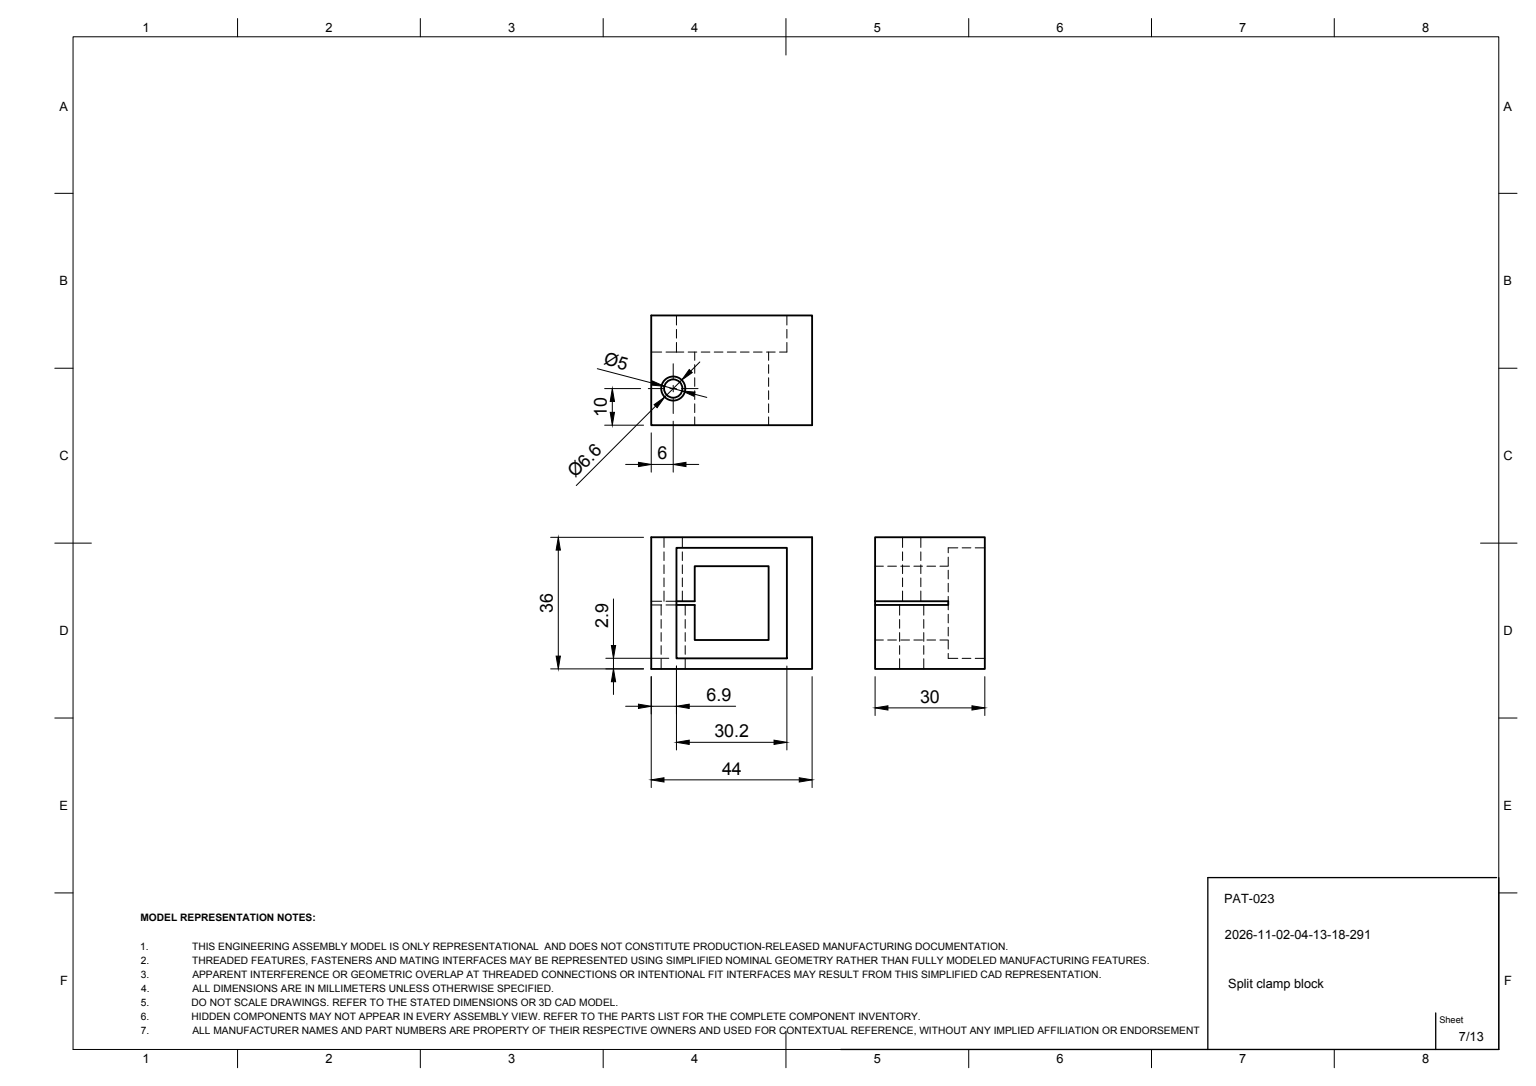
ISO-10303-21;
HEADER;
/* Generated by software containing ST-Developer
 * from STEP Tools, Inc. (www.steptools.com) 
 */

FILE_DESCRIPTION(
/* description */ ('PAT-023'),
/* implementation_level */ '2;1');

FILE_NAME(
/* name */ 'Split clamp block.step',
/* time_stamp */ '2026-10-29T15:47:46-07:00',
/* author */ (''),
/* organization */ (''),
/* preprocessor_version */ 'ST-DEVELOPER v20.2',
/* originating_system */ 'Autodesk Translation Framework v15.17.0.0',
/* authorisation */ '');

FILE_SCHEMA (('AUTOMOTIVE_DESIGN { 1 0 10303 214 3 1 1 }'));
ENDSEC;

DATA;
#10=MECHANICAL_DESIGN_GEOMETRIC_PRESENTATION_REPRESENTATION('',(#86),#3773);
#70=SHAPE_REPRESENTATION_RELATIONSHIP('SRR','None',#3817,#78);
#78=ADVANCED_BREP_SHAPE_REPRESENTATION('',(#94),#3765);
#86=STYLED_ITEM('',(#3925),#94);
#94=MANIFOLD_SOLID_BREP('Body1',#2239);
#104=FACE_BOUND('',#361,.T.);
#105=FACE_BOUND('',#363,.T.);
#106=FACE_BOUND('',#378,.T.);
#107=FACE_BOUND('',#380,.T.);
#108=FACE_BOUND('',#383,.T.);
#131=PLANE('',#2364);
#132=PLANE('',#2365);
#133=PLANE('',#2366);
#134=PLANE('',#2367);
#135=PLANE('',#2368);
#136=PLANE('',#2369);
#137=PLANE('',#2370);
#138=PLANE('',#2371);
#139=PLANE('',#2372);
#140=PLANE('',#2373);
#141=PLANE('',#2374);
#142=PLANE('',#2375);
#143=PLANE('',#2376);
#144=PLANE('',#2377);
#145=PLANE('',#2378);
#146=PLANE('',#2379);
#147=PLANE('',#2380);
#148=PLANE('',#2381);
#149=PLANE('',#2382);
#235=FACE_OUTER_BOUND('',#358,.T.);
#236=FACE_OUTER_BOUND('',#359,.T.);
#237=FACE_OUTER_BOUND('',#360,.T.);
#238=FACE_OUTER_BOUND('',#362,.T.);
#239=FACE_OUTER_BOUND('',#364,.T.);
#240=FACE_OUTER_BOUND('',#365,.T.);
#241=FACE_OUTER_BOUND('',#366,.T.);
#242=FACE_OUTER_BOUND('',#367,.T.);
#243=FACE_OUTER_BOUND('',#368,.T.);
#244=FACE_OUTER_BOUND('',#369,.T.);
#245=FACE_OUTER_BOUND('',#370,.T.);
#246=FACE_OUTER_BOUND('',#371,.T.);
#247=FACE_OUTER_BOUND('',#372,.T.);
#248=FACE_OUTER_BOUND('',#373,.T.);
#249=FACE_OUTER_BOUND('',#374,.T.);
#250=FACE_OUTER_BOUND('',#375,.T.);
#251=FACE_OUTER_BOUND('',#376,.T.);
#252=FACE_OUTER_BOUND('',#377,.T.);
#253=FACE_OUTER_BOUND('',#379,.T.);
#254=FACE_OUTER_BOUND('',#381,.T.);
#255=FACE_OUTER_BOUND('',#382,.T.);
#358=EDGE_LOOP('',(#1595,#1596,#1597,#1598));
#359=EDGE_LOOP('',(#1599,#1600,#1601,#1602));
#360=EDGE_LOOP('',(#1603,#1604,#1605,#1606,#1607));
#361=EDGE_LOOP('',(#1608));
#362=EDGE_LOOP('',(#1609,#1610,#1611,#1612,#1613));
#363=EDGE_LOOP('',(#1614));
#364=EDGE_LOOP('',(#1615,#1616,#1617,#1618));
#365=EDGE_LOOP('',(#1619,#1620,#1621,#1622,#1623,#1624,#1625,#1626,#1627,
#1628,#1629,#1630));
#366=EDGE_LOOP('',(#1631,#1632,#1633,#1634));
#367=EDGE_LOOP('',(#1635,#1636,#1637,#1638));
#368=EDGE_LOOP('',(#1639,#1640,#1641,#1642,#1643,#1644,#1645,#1646));
#369=EDGE_LOOP('',(#1647,#1648,#1649,#1650,#1651,#1652,#1653,#1654,#1655,
#1656,#1657,#1658));
#370=EDGE_LOOP('',(#1659,#1660,#1661,#1662));
#371=EDGE_LOOP('',(#1663,#1664,#1665,#1666));
#372=EDGE_LOOP('',(#1667,#1668,#1669,#1670));
#373=EDGE_LOOP('',(#1671,#1672,#1673,#1674));
#374=EDGE_LOOP('',(#1675,#1676,#1677,#1678,#1679,#1680));
#375=EDGE_LOOP('',(#1681,#1682,#1683,#1684));
#376=EDGE_LOOP('',(#1685,#1686,#1687,#1688));
#377=EDGE_LOOP('',(#1689,#1690,#1691,#1692));
#378=EDGE_LOOP('',(#1693));
#379=EDGE_LOOP('',(#1694,#1695,#1696,#1697));
#380=EDGE_LOOP('',(#1698));
#381=EDGE_LOOP('',(#1699,#1700,#1701,#1702));
#382=EDGE_LOOP('',(#1703,#1704,#1705,#1706));
#383=EDGE_LOOP('',(#1707,#1708,#1709,#1710));
#508=LINE('',#3193,#772);
#509=LINE('',#3199,#773);
#510=LINE('',#3204,#774);
#511=LINE('',#3206,#775);
#512=LINE('',#3208,#776);
#513=LINE('',#3210,#777);
#514=LINE('',#3211,#778);
#515=LINE('',#3215,#779);
#516=LINE('',#3217,#780);
#517=LINE('',#3219,#781);
#518=LINE('',#3221,#782);
#519=LINE('',#3222,#783);
#520=LINE('',#3224,#784);
#521=LINE('',#3225,#785);
#522=LINE('',#3228,#786);
#523=LINE('',#3230,#787);
#524=LINE('',#3232,#788);
#525=LINE('',#3234,#789);
#526=LINE('',#3235,#790);
#527=LINE('',#3237,#791);
#528=LINE('',#3239,#792);
#529=LINE('',#3241,#793);
#530=LINE('',#3243,#794);
#531=LINE('',#3244,#795);
#532=LINE('',#3247,#796);
#533=LINE('',#3248,#797);
#534=LINE('',#3251,#798);
#535=LINE('',#3252,#799);
#536=LINE('',#3255,#800);
#537=LINE('',#3257,#801);
#538=LINE('',#3259,#802);
#539=LINE('',#3261,#803);
#540=LINE('',#3262,#804);
#541=LINE('',#3265,#805);
#542=LINE('',#3267,#806);
#543=LINE('',#3268,#807);
#544=LINE('',#3270,#808);
#545=LINE('',#3272,#809);
#546=LINE('',#3273,#810);
#547=LINE('',#3275,#811);
#548=LINE('',#3277,#812);
#549=LINE('',#3282,#813);
#550=LINE('',#3283,#814);
#551=LINE('',#3284,#815);
#552=LINE('',#3287,#816);
#553=LINE('',#3288,#817);
#554=LINE('',#3291,#818);
#555=LINE('',#3292,#819);
#556=LINE('',#3294,#820);
#557=LINE('',#3297,#821);
#558=LINE('',#3298,#822);
#559=LINE('',#3301,#823);
#560=LINE('',#3302,#824);
#561=LINE('',#3304,#825);
#772=VECTOR('',#2591,0.25);
#773=VECTOR('',#2598,0.33);
#774=VECTOR('',#2603,1.);
#775=VECTOR('',#2604,1.);
#776=VECTOR('',#2605,1.);
#777=VECTOR('',#2606,1.);
#778=VECTOR('',#2607,1.);
#779=VECTOR('',#2610,1.);
#780=VECTOR('',#2611,1.);
#781=VECTOR('',#2612,1.);
#782=VECTOR('',#2613,1.);
#783=VECTOR('',#2614,1.);
#784=VECTOR('',#2617,1.);
#785=VECTOR('',#2618,1.);
#786=VECTOR('',#2621,1.);
#787=VECTOR('',#2622,1.);
#788=VECTOR('',#2623,1.);
#789=VECTOR('',#2624,1.);
#790=VECTOR('',#2625,1.);
#791=VECTOR('',#2626,1.);
#792=VECTOR('',#2627,1.);
#793=VECTOR('',#2628,1.);
#794=VECTOR('',#2629,1.);
#795=VECTOR('',#2630,1.);
#796=VECTOR('',#2633,1.);
#797=VECTOR('',#2634,1.);
#798=VECTOR('',#2637,1.);
#799=VECTOR('',#2638,1.);
#800=VECTOR('',#2641,1.);
#801=VECTOR('',#2642,1.);
#802=VECTOR('',#2643,1.);
#803=VECTOR('',#2644,1.);
#804=VECTOR('',#2645,1.);
#805=VECTOR('',#2648,1.);
#806=VECTOR('',#2649,1.);
#807=VECTOR('',#2650,1.);
#808=VECTOR('',#2651,1.);
#809=VECTOR('',#2652,1.);
#810=VECTOR('',#2653,1.);
#811=VECTOR('',#2656,1.);
#812=VECTOR('',#2659,1.);
#813=VECTOR('',#2664,1.);
#814=VECTOR('',#2665,1.);
#815=VECTOR('',#2666,1.);
#816=VECTOR('',#2669,1.);
#817=VECTOR('',#2670,1.);
#818=VECTOR('',#2673,1.);
#819=VECTOR('',#2674,1.);
#820=VECTOR('',#2677,1.);
#821=VECTOR('',#2680,1.);
#822=VECTOR('',#2681,1.);
#823=VECTOR('',#2684,1.);
#824=VECTOR('',#2685,1.);
#825=VECTOR('',#2688,1.);
#1001=CIRCLE('',#2359,0.25);
#1002=CIRCLE('',#2360,0.25);
#1003=CIRCLE('',#2362,0.33);
#1004=CIRCLE('',#2363,0.33);
#1051=VERTEX_POINT('',#3190);
#1052=VERTEX_POINT('',#3192);
#1053=VERTEX_POINT('',#3196);
#1054=VERTEX_POINT('',#3198);
#1055=VERTEX_POINT('',#3202);
#1056=VERTEX_POINT('',#3203);
#1057=VERTEX_POINT('',#3205);
#1058=VERTEX_POINT('',#3207);
#1059=VERTEX_POINT('',#3209);
#1060=VERTEX_POINT('',#3213);
#1061=VERTEX_POINT('',#3214);
#1062=VERTEX_POINT('',#3216);
#1063=VERTEX_POINT('',#3218);
#1064=VERTEX_POINT('',#3220);
#1065=VERTEX_POINT('',#3227);
#1066=VERTEX_POINT('',#3229);
#1067=VERTEX_POINT('',#3231);
#1068=VERTEX_POINT('',#3233);
#1069=VERTEX_POINT('',#3236);
#1070=VERTEX_POINT('',#3238);
#1071=VERTEX_POINT('',#3240);
#1072=VERTEX_POINT('',#3242);
#1073=VERTEX_POINT('',#3246);
#1074=VERTEX_POINT('',#3250);
#1075=VERTEX_POINT('',#3254);
#1076=VERTEX_POINT('',#3256);
#1077=VERTEX_POINT('',#3258);
#1078=VERTEX_POINT('',#3260);
#1079=VERTEX_POINT('',#3264);
#1080=VERTEX_POINT('',#3266);
#1081=VERTEX_POINT('',#3269);
#1082=VERTEX_POINT('',#3271);
#1083=VERTEX_POINT('',#3280);
#1084=VERTEX_POINT('',#3281);
#1085=VERTEX_POINT('',#3286);
#1086=VERTEX_POINT('',#3290);
#1087=VERTEX_POINT('',#3296);
#1088=VERTEX_POINT('',#3300);
#1260=EDGE_CURVE('',#1051,#1051,#1001,.T.);
#1261=EDGE_CURVE('',#1051,#1052,#508,.T.);
#1262=EDGE_CURVE('',#1052,#1052,#1002,.T.);
#1263=EDGE_CURVE('',#1053,#1053,#1003,.T.);
#1264=EDGE_CURVE('',#1053,#1054,#509,.T.);
#1265=EDGE_CURVE('',#1054,#1054,#1004,.T.);
#1266=EDGE_CURVE('',#1055,#1056,#510,.T.);
#1267=EDGE_CURVE('',#1057,#1055,#511,.T.);
#1268=EDGE_CURVE('',#1058,#1057,#512,.T.);
#1269=EDGE_CURVE('',#1059,#1058,#513,.T.);
#1270=EDGE_CURVE('',#1056,#1059,#514,.T.);
#1271=EDGE_CURVE('',#1060,#1061,#515,.T.);
#1272=EDGE_CURVE('',#1062,#1060,#516,.T.);
#1273=EDGE_CURVE('',#1063,#1062,#517,.T.);
#1274=EDGE_CURVE('',#1064,#1063,#518,.T.);
#1275=EDGE_CURVE('',#1061,#1064,#519,.T.);
#1276=EDGE_CURVE('',#1064,#1057,#520,.T.);
#1277=EDGE_CURVE('',#1058,#1063,#521,.T.);
#1278=EDGE_CURVE('',#1055,#1065,#522,.T.);
#1279=EDGE_CURVE('',#1065,#1066,#523,.T.);
#1280=EDGE_CURVE('',#1066,#1067,#524,.T.);
#1281=EDGE_CURVE('',#1067,#1068,#525,.T.);
#1282=EDGE_CURVE('',#1068,#1061,#526,.T.);
#1283=EDGE_CURVE('',#1069,#1064,#527,.T.);
#1284=EDGE_CURVE('',#1070,#1069,#528,.T.);
#1285=EDGE_CURVE('',#1071,#1070,#529,.T.);
#1286=EDGE_CURVE('',#1072,#1071,#530,.T.);
#1287=EDGE_CURVE('',#1057,#1072,#531,.T.);
#1288=EDGE_CURVE('',#1068,#1073,#532,.T.);
#1289=EDGE_CURVE('',#1060,#1073,#533,.T.);
#1290=EDGE_CURVE('',#1074,#1056,#534,.T.);
#1291=EDGE_CURVE('',#1065,#1074,#535,.T.);
#1292=EDGE_CURVE('',#1075,#1062,#536,.T.);
#1293=EDGE_CURVE('',#1076,#1075,#537,.T.);
#1294=EDGE_CURVE('',#1076,#1077,#538,.T.);
#1295=EDGE_CURVE('',#1077,#1078,#539,.T.);
#1296=EDGE_CURVE('',#1059,#1078,#540,.T.);
#1297=EDGE_CURVE('',#1078,#1079,#541,.T.);
#1298=EDGE_CURVE('',#1079,#1080,#542,.T.);
#1299=EDGE_CURVE('',#1080,#1075,#543,.T.);
#1300=EDGE_CURVE('',#1073,#1081,#544,.T.);
#1301=EDGE_CURVE('',#1081,#1082,#545,.T.);
#1302=EDGE_CURVE('',#1082,#1074,#546,.T.);
#1303=EDGE_CURVE('',#1067,#1081,#547,.T.);
#1304=EDGE_CURVE('',#1066,#1082,#548,.T.);
#1305=EDGE_CURVE('',#1083,#1084,#549,.T.);
#1306=EDGE_CURVE('',#1083,#1070,#550,.T.);
#1307=EDGE_CURVE('',#1084,#1069,#551,.T.);
#1308=EDGE_CURVE('',#1084,#1085,#552,.T.);
#1309=EDGE_CURVE('',#1085,#1072,#553,.T.);
#1310=EDGE_CURVE('',#1085,#1086,#554,.T.);
#1311=EDGE_CURVE('',#1086,#1071,#555,.T.);
#1312=EDGE_CURVE('',#1086,#1083,#556,.T.);
#1313=EDGE_CURVE('',#1077,#1087,#557,.T.);
#1314=EDGE_CURVE('',#1087,#1079,#558,.T.);
#1315=EDGE_CURVE('',#1088,#1076,#559,.T.);
#1316=EDGE_CURVE('',#1088,#1080,#560,.T.);
#1317=EDGE_CURVE('',#1087,#1088,#561,.T.);
#1595=ORIENTED_EDGE('',*,*,#1260,.F.);
#1596=ORIENTED_EDGE('',*,*,#1261,.T.);
#1597=ORIENTED_EDGE('',*,*,#1262,.F.);
#1598=ORIENTED_EDGE('',*,*,#1261,.F.);
#1599=ORIENTED_EDGE('',*,*,#1263,.F.);
#1600=ORIENTED_EDGE('',*,*,#1264,.T.);
#1601=ORIENTED_EDGE('',*,*,#1265,.F.);
#1602=ORIENTED_EDGE('',*,*,#1264,.F.);
#1603=ORIENTED_EDGE('',*,*,#1266,.F.);
#1604=ORIENTED_EDGE('',*,*,#1267,.F.);
#1605=ORIENTED_EDGE('',*,*,#1268,.F.);
#1606=ORIENTED_EDGE('',*,*,#1269,.F.);
#1607=ORIENTED_EDGE('',*,*,#1270,.F.);
#1608=ORIENTED_EDGE('',*,*,#1260,.T.);
#1609=ORIENTED_EDGE('',*,*,#1271,.F.);
#1610=ORIENTED_EDGE('',*,*,#1272,.F.);
#1611=ORIENTED_EDGE('',*,*,#1273,.F.);
#1612=ORIENTED_EDGE('',*,*,#1274,.F.);
#1613=ORIENTED_EDGE('',*,*,#1275,.F.);
#1614=ORIENTED_EDGE('',*,*,#1265,.T.);
#1615=ORIENTED_EDGE('',*,*,#1276,.F.);
#1616=ORIENTED_EDGE('',*,*,#1274,.T.);
#1617=ORIENTED_EDGE('',*,*,#1277,.F.);
#1618=ORIENTED_EDGE('',*,*,#1268,.T.);
#1619=ORIENTED_EDGE('',*,*,#1267,.T.);
#1620=ORIENTED_EDGE('',*,*,#1278,.T.);
#1621=ORIENTED_EDGE('',*,*,#1279,.T.);
#1622=ORIENTED_EDGE('',*,*,#1280,.T.);
#1623=ORIENTED_EDGE('',*,*,#1281,.T.);
#1624=ORIENTED_EDGE('',*,*,#1282,.T.);
#1625=ORIENTED_EDGE('',*,*,#1275,.T.);
#1626=ORIENTED_EDGE('',*,*,#1283,.F.);
#1627=ORIENTED_EDGE('',*,*,#1284,.F.);
#1628=ORIENTED_EDGE('',*,*,#1285,.F.);
#1629=ORIENTED_EDGE('',*,*,#1286,.F.);
#1630=ORIENTED_EDGE('',*,*,#1287,.F.);
#1631=ORIENTED_EDGE('',*,*,#1271,.T.);
#1632=ORIENTED_EDGE('',*,*,#1282,.F.);
#1633=ORIENTED_EDGE('',*,*,#1288,.T.);
#1634=ORIENTED_EDGE('',*,*,#1289,.F.);
#1635=ORIENTED_EDGE('',*,*,#1266,.T.);
#1636=ORIENTED_EDGE('',*,*,#1290,.F.);
#1637=ORIENTED_EDGE('',*,*,#1291,.F.);
#1638=ORIENTED_EDGE('',*,*,#1278,.F.);
#1639=ORIENTED_EDGE('',*,*,#1269,.T.);
#1640=ORIENTED_EDGE('',*,*,#1277,.T.);
#1641=ORIENTED_EDGE('',*,*,#1273,.T.);
#1642=ORIENTED_EDGE('',*,*,#1292,.F.);
#1643=ORIENTED_EDGE('',*,*,#1293,.F.);
#1644=ORIENTED_EDGE('',*,*,#1294,.T.);
#1645=ORIENTED_EDGE('',*,*,#1295,.T.);
#1646=ORIENTED_EDGE('',*,*,#1296,.F.);
#1647=ORIENTED_EDGE('',*,*,#1270,.T.);
#1648=ORIENTED_EDGE('',*,*,#1296,.T.);
#1649=ORIENTED_EDGE('',*,*,#1297,.T.);
#1650=ORIENTED_EDGE('',*,*,#1298,.T.);
#1651=ORIENTED_EDGE('',*,*,#1299,.T.);
#1652=ORIENTED_EDGE('',*,*,#1292,.T.);
#1653=ORIENTED_EDGE('',*,*,#1272,.T.);
#1654=ORIENTED_EDGE('',*,*,#1289,.T.);
#1655=ORIENTED_EDGE('',*,*,#1300,.T.);
#1656=ORIENTED_EDGE('',*,*,#1301,.T.);
#1657=ORIENTED_EDGE('',*,*,#1302,.T.);
#1658=ORIENTED_EDGE('',*,*,#1290,.T.);
#1659=ORIENTED_EDGE('',*,*,#1281,.F.);
#1660=ORIENTED_EDGE('',*,*,#1303,.T.);
#1661=ORIENTED_EDGE('',*,*,#1300,.F.);
#1662=ORIENTED_EDGE('',*,*,#1288,.F.);
#1663=ORIENTED_EDGE('',*,*,#1279,.F.);
#1664=ORIENTED_EDGE('',*,*,#1291,.T.);
#1665=ORIENTED_EDGE('',*,*,#1302,.F.);
#1666=ORIENTED_EDGE('',*,*,#1304,.F.);
#1667=ORIENTED_EDGE('',*,*,#1280,.F.);
#1668=ORIENTED_EDGE('',*,*,#1304,.T.);
#1669=ORIENTED_EDGE('',*,*,#1301,.F.);
#1670=ORIENTED_EDGE('',*,*,#1303,.F.);
#1671=ORIENTED_EDGE('',*,*,#1305,.F.);
#1672=ORIENTED_EDGE('',*,*,#1306,.T.);
#1673=ORIENTED_EDGE('',*,*,#1284,.T.);
#1674=ORIENTED_EDGE('',*,*,#1307,.F.);
#1675=ORIENTED_EDGE('',*,*,#1308,.F.);
#1676=ORIENTED_EDGE('',*,*,#1307,.T.);
#1677=ORIENTED_EDGE('',*,*,#1283,.T.);
#1678=ORIENTED_EDGE('',*,*,#1276,.T.);
#1679=ORIENTED_EDGE('',*,*,#1287,.T.);
#1680=ORIENTED_EDGE('',*,*,#1309,.F.);
#1681=ORIENTED_EDGE('',*,*,#1310,.F.);
#1682=ORIENTED_EDGE('',*,*,#1309,.T.);
#1683=ORIENTED_EDGE('',*,*,#1286,.T.);
#1684=ORIENTED_EDGE('',*,*,#1311,.F.);
#1685=ORIENTED_EDGE('',*,*,#1312,.F.);
#1686=ORIENTED_EDGE('',*,*,#1311,.T.);
#1687=ORIENTED_EDGE('',*,*,#1285,.T.);
#1688=ORIENTED_EDGE('',*,*,#1306,.F.);
#1689=ORIENTED_EDGE('',*,*,#1313,.T.);
#1690=ORIENTED_EDGE('',*,*,#1314,.T.);
#1691=ORIENTED_EDGE('',*,*,#1297,.F.);
#1692=ORIENTED_EDGE('',*,*,#1295,.F.);
#1693=ORIENTED_EDGE('',*,*,#1262,.T.);
#1694=ORIENTED_EDGE('',*,*,#1315,.T.);
#1695=ORIENTED_EDGE('',*,*,#1293,.T.);
#1696=ORIENTED_EDGE('',*,*,#1299,.F.);
#1697=ORIENTED_EDGE('',*,*,#1316,.F.);
#1698=ORIENTED_EDGE('',*,*,#1263,.T.);
#1699=ORIENTED_EDGE('',*,*,#1317,.T.);
#1700=ORIENTED_EDGE('',*,*,#1316,.T.);
#1701=ORIENTED_EDGE('',*,*,#1298,.F.);
#1702=ORIENTED_EDGE('',*,*,#1314,.F.);
#1703=ORIENTED_EDGE('',*,*,#1317,.F.);
#1704=ORIENTED_EDGE('',*,*,#1313,.F.);
#1705=ORIENTED_EDGE('',*,*,#1294,.F.);
#1706=ORIENTED_EDGE('',*,*,#1315,.F.);
#1707=ORIENTED_EDGE('',*,*,#1310,.T.);
#1708=ORIENTED_EDGE('',*,*,#1312,.T.);
#1709=ORIENTED_EDGE('',*,*,#1305,.T.);
#1710=ORIENTED_EDGE('',*,*,#1308,.T.);
#2110=CYLINDRICAL_SURFACE('',#2358,0.25);
#2111=CYLINDRICAL_SURFACE('',#2361,0.33);
#2135=ADVANCED_FACE('',(#235),#2110,.F.);
#2136=ADVANCED_FACE('',(#236),#2111,.F.);
#2137=ADVANCED_FACE('',(#237,#104),#131,.F.);
#2138=ADVANCED_FACE('',(#238,#105),#132,.F.);
#2139=ADVANCED_FACE('',(#239),#133,.T.);
#2140=ADVANCED_FACE('',(#240),#134,.F.);
#2141=ADVANCED_FACE('',(#241),#135,.F.);
#2142=ADVANCED_FACE('',(#242),#136,.F.);
#2143=ADVANCED_FACE('',(#243),#137,.T.);
#2144=ADVANCED_FACE('',(#244),#138,.T.);
#2145=ADVANCED_FACE('',(#245),#139,.F.);
#2146=ADVANCED_FACE('',(#246),#140,.F.);
#2147=ADVANCED_FACE('',(#247),#141,.F.);
#2148=ADVANCED_FACE('',(#248),#142,.F.);
#2149=ADVANCED_FACE('',(#249),#143,.F.);
#2150=ADVANCED_FACE('',(#250),#144,.F.);
#2151=ADVANCED_FACE('',(#251),#145,.F.);
#2152=ADVANCED_FACE('',(#252,#106),#146,.T.);
#2153=ADVANCED_FACE('',(#253,#107),#147,.T.);
#2154=ADVANCED_FACE('',(#254),#148,.T.);
#2155=ADVANCED_FACE('',(#255,#108),#149,.F.);
#2239=CLOSED_SHELL('',(#2135,#2136,#2137,#2138,#2139,#2140,#2141,#2142,
#2143,#2144,#2145,#2146,#2147,#2148,#2149,#2150,#2151,#2152,#2153,#2154,
#2155));
#2357=AXIS2_PLACEMENT_3D('',#3188,#2585,#2586);
#2358=AXIS2_PLACEMENT_3D('',#3189,#2587,#2588);
#2359=AXIS2_PLACEMENT_3D('',#3191,#2589,#2590);
#2360=AXIS2_PLACEMENT_3D('',#3194,#2592,#2593);
#2361=AXIS2_PLACEMENT_3D('',#3195,#2594,#2595);
#2362=AXIS2_PLACEMENT_3D('',#3197,#2596,#2597);
#2363=AXIS2_PLACEMENT_3D('',#3200,#2599,#2600);
#2364=AXIS2_PLACEMENT_3D('',#3201,#2601,#2602);
#2365=AXIS2_PLACEMENT_3D('',#3212,#2608,#2609);
#2366=AXIS2_PLACEMENT_3D('',#3223,#2615,#2616);
#2367=AXIS2_PLACEMENT_3D('',#3226,#2619,#2620);
#2368=AXIS2_PLACEMENT_3D('',#3245,#2631,#2632);
#2369=AXIS2_PLACEMENT_3D('',#3249,#2635,#2636);
#2370=AXIS2_PLACEMENT_3D('',#3253,#2639,#2640);
#2371=AXIS2_PLACEMENT_3D('',#3263,#2646,#2647);
#2372=AXIS2_PLACEMENT_3D('',#3274,#2654,#2655);
#2373=AXIS2_PLACEMENT_3D('',#3276,#2657,#2658);
#2374=AXIS2_PLACEMENT_3D('',#3278,#2660,#2661);
#2375=AXIS2_PLACEMENT_3D('',#3279,#2662,#2663);
#2376=AXIS2_PLACEMENT_3D('',#3285,#2667,#2668);
#2377=AXIS2_PLACEMENT_3D('',#3289,#2671,#2672);
#2378=AXIS2_PLACEMENT_3D('',#3293,#2675,#2676);
#2379=AXIS2_PLACEMENT_3D('',#3295,#2678,#2679);
#2380=AXIS2_PLACEMENT_3D('',#3299,#2682,#2683);
#2381=AXIS2_PLACEMENT_3D('',#3303,#2686,#2687);
#2382=AXIS2_PLACEMENT_3D('',#3305,#2689,#2690);
#2585=DIRECTION('axis',(0.,0.,1.));
#2586=DIRECTION('refdir',(1.,0.,0.));
#2587=DIRECTION('center_axis',(0.,1.,0.));
#2588=DIRECTION('ref_axis',(1.,0.,0.));
#2589=DIRECTION('center_axis',(0.,1.,0.));
#2590=DIRECTION('ref_axis',(1.,0.,0.));
#2591=DIRECTION('',(0.,1.,0.));
#2592=DIRECTION('center_axis',(0.,-1.,0.));
#2593=DIRECTION('ref_axis',(1.,0.,0.));
#2594=DIRECTION('center_axis',(0.,1.,0.));
#2595=DIRECTION('ref_axis',(1.,0.,0.));
#2596=DIRECTION('center_axis',(0.,1.,0.));
#2597=DIRECTION('ref_axis',(1.,0.,0.));
#2598=DIRECTION('',(0.,1.,0.));
#2599=DIRECTION('center_axis',(0.,-1.,0.));
#2600=DIRECTION('ref_axis',(1.,0.,0.));
#2601=DIRECTION('center_axis',(0.,1.,0.));
#2602=DIRECTION('ref_axis',(-1.,0.,0.));
#2603=DIRECTION('',(0.,0.,1.));
#2604=DIRECTION('',(-1.,0.,0.));
#2605=DIRECTION('',(-1.,0.,0.));
#2606=DIRECTION('',(0.,0.,-1.));
#2607=DIRECTION('',(1.,0.,0.));
#2608=DIRECTION('center_axis',(0.,-1.,0.));
#2609=DIRECTION('ref_axis',(1.,0.,0.));
#2610=DIRECTION('',(0.,0.,-1.));
#2611=DIRECTION('',(-1.,0.,0.));
#2612=DIRECTION('',(0.,0.,1.));
#2613=DIRECTION('',(1.,0.,0.));
#2614=DIRECTION('',(1.,0.,0.));
#2615=DIRECTION('center_axis',(0.,0.,1.));
#2616=DIRECTION('ref_axis',(1.,0.,0.));
#2617=DIRECTION('',(0.,1.,0.));
#2618=DIRECTION('',(0.,-1.,0.));
#2619=DIRECTION('center_axis',(0.,0.,1.));
#2620=DIRECTION('ref_axis',(1.,0.,0.));
#2621=DIRECTION('',(0.,1.,0.));
#2622=DIRECTION('',(-1.,0.,0.));
#2623=DIRECTION('',(0.,-1.,0.));
#2624=DIRECTION('',(1.,0.,0.));
#2625=DIRECTION('',(0.,1.,0.));
#2626=DIRECTION('',(0.,1.,0.));
#2627=DIRECTION('',(1.,0.,0.));
#2628=DIRECTION('',(0.,-1.,0.));
#2629=DIRECTION('',(-1.,0.,0.));
#2630=DIRECTION('',(0.,1.,0.));
#2631=DIRECTION('center_axis',(1.,0.,0.));
#2632=DIRECTION('ref_axis',(0.,1.,0.));
#2633=DIRECTION('',(0.,0.,1.));
#2634=DIRECTION('',(0.,-1.,0.));
#2635=DIRECTION('center_axis',(1.,0.,0.));
#2636=DIRECTION('ref_axis',(0.,1.,0.));
#2637=DIRECTION('',(0.,-1.,0.));
#2638=DIRECTION('',(0.,0.,1.));
#2639=DIRECTION('center_axis',(1.,0.,0.));
#2640=DIRECTION('ref_axis',(0.,1.,0.));
#2641=DIRECTION('',(0.,1.,0.));
#2642=DIRECTION('',(0.,0.,1.));
#2643=DIRECTION('',(0.,1.,0.));
#2644=DIRECTION('',(0.,0.,1.));
#2645=DIRECTION('',(0.,1.,0.));
#2646=DIRECTION('center_axis',(0.,0.,1.));
#2647=DIRECTION('ref_axis',(1.,0.,0.));
#2648=DIRECTION('',(-1.,0.,0.));
#2649=DIRECTION('',(0.,-1.,0.));
#2650=DIRECTION('',(1.,0.,0.));
#2651=DIRECTION('',(-1.,0.,0.));
#2652=DIRECTION('',(0.,1.,0.));
#2653=DIRECTION('',(1.,0.,0.));
#2654=DIRECTION('center_axis',(0.,-1.,0.));
#2655=DIRECTION('ref_axis',(1.,0.,0.));
#2656=DIRECTION('',(0.,0.,1.));
#2657=DIRECTION('center_axis',(0.,1.,0.));
#2658=DIRECTION('ref_axis',(-1.,0.,0.));
#2659=DIRECTION('',(0.,0.,1.));
#2660=DIRECTION('center_axis',(-1.,0.,0.));
#2661=DIRECTION('ref_axis',(0.,-1.,0.));
#2662=DIRECTION('center_axis',(0.,-1.,0.));
#2663=DIRECTION('ref_axis',(1.,0.,0.));
#2664=DIRECTION('',(1.,0.,0.));
#2665=DIRECTION('',(0.,0.,1.));
#2666=DIRECTION('',(0.,0.,1.));
#2667=DIRECTION('center_axis',(1.,0.,0.));
#2668=DIRECTION('ref_axis',(0.,1.,0.));
#2669=DIRECTION('',(0.,1.,0.));
#2670=DIRECTION('',(0.,0.,1.));
#2671=DIRECTION('center_axis',(0.,1.,0.));
#2672=DIRECTION('ref_axis',(-1.,0.,0.));
#2673=DIRECTION('',(-1.,0.,0.));
#2674=DIRECTION('',(0.,0.,1.));
#2675=DIRECTION('center_axis',(-1.,0.,0.));
#2676=DIRECTION('ref_axis',(0.,-1.,0.));
#2677=DIRECTION('',(0.,-1.,0.));
#2678=DIRECTION('center_axis',(0.,1.,0.));
#2679=DIRECTION('ref_axis',(-1.,0.,0.));
#2680=DIRECTION('',(-1.,0.,0.));
#2681=DIRECTION('',(0.,0.,1.));
#2682=DIRECTION('center_axis',(0.,-1.,0.));
#2683=DIRECTION('ref_axis',(1.,0.,0.));
#2684=DIRECTION('',(1.,0.,0.));
#2685=DIRECTION('',(0.,0.,1.));
#2686=DIRECTION('center_axis',(-1.,0.,0.));
#2687=DIRECTION('ref_axis',(0.,-1.,0.));
#2688=DIRECTION('',(0.,-1.,0.));
#2689=DIRECTION('center_axis',(0.,0.,1.));
#2690=DIRECTION('ref_axis',(1.,0.,0.));
#3188=CARTESIAN_POINT('',(0.,0.,0.));
#3189=CARTESIAN_POINT('Origin',(1.6,0.05,28.));
#3190=CARTESIAN_POINT('',(1.35,0.05,28.));
#3191=CARTESIAN_POINT('Origin',(1.6,0.05,28.));
#3192=CARTESIAN_POINT('',(1.35,1.8,28.));
#3193=CARTESIAN_POINT('',(1.35,0.05,28.));
#3194=CARTESIAN_POINT('Origin',(1.6,1.8,28.));
#3195=CARTESIAN_POINT('Origin',(1.6,-1.9,28.));
#3196=CARTESIAN_POINT('',(1.27,-1.8,28.));
#3197=CARTESIAN_POINT('Origin',(1.6,-1.8,28.));
#3198=CARTESIAN_POINT('',(1.27,-0.05,28.));
#3199=CARTESIAN_POINT('',(1.27,-1.9,28.));
#3200=CARTESIAN_POINT('Origin',(1.6,-0.05,28.));
#3201=CARTESIAN_POINT('Origin',(2.3,0.05,27.));
#3202=CARTESIAN_POINT('',(1.01,0.05,27.));
#3203=CARTESIAN_POINT('',(1.01,0.05,29.));
#3204=CARTESIAN_POINT('',(1.01,0.05,26.95));
#3205=CARTESIAN_POINT('',(1.51,0.05,27.));
#3206=CARTESIAN_POINT('',(1.15,0.05,27.));
#3207=CARTESIAN_POINT('',(2.2,0.05,27.));
#3208=CARTESIAN_POINT('',(2.3,0.05,27.));
#3209=CARTESIAN_POINT('',(2.2,0.05,29.));
#3210=CARTESIAN_POINT('',(2.2,0.05,26.5));
#3211=CARTESIAN_POINT('',(1.15,0.05,29.));
#3212=CARTESIAN_POINT('Origin',(0.,-0.05,27.));
#3213=CARTESIAN_POINT('',(1.01,-0.05,29.));
#3214=CARTESIAN_POINT('',(1.01,-0.05,27.));
#3215=CARTESIAN_POINT('',(1.01,-0.05,26.95));
#3216=CARTESIAN_POINT('',(2.2,-0.05,29.));
#3217=CARTESIAN_POINT('',(0.,-0.05,29.));
#3218=CARTESIAN_POINT('',(2.2,-0.05,27.));
#3219=CARTESIAN_POINT('',(2.2,-0.05,26.5));
#3220=CARTESIAN_POINT('',(1.51,-0.05,27.));
#3221=CARTESIAN_POINT('',(0.,-0.05,27.));
#3222=CARTESIAN_POINT('',(0.,-0.05,27.));
#3223=CARTESIAN_POINT('Origin',(1.15,0.,27.));
#3224=CARTESIAN_POINT('',(1.51,-1.51,27.));
#3225=CARTESIAN_POINT('',(2.2,-0.9,27.));
#3226=CARTESIAN_POINT('Origin',(0.,0.,27.));
#3227=CARTESIAN_POINT('',(1.01,1.01,27.));
#3228=CARTESIAN_POINT('',(1.01,-0.505,27.));
#3229=CARTESIAN_POINT('',(-1.01,1.01,27.));
#3230=CARTESIAN_POINT('',(0.505,1.01,27.));
#3231=CARTESIAN_POINT('',(-1.01,-1.01,27.));
#3232=CARTESIAN_POINT('',(-1.01,0.505,27.));
#3233=CARTESIAN_POINT('',(1.01,-1.01,27.));
#3234=CARTESIAN_POINT('',(-0.505,-1.01,27.));
#3235=CARTESIAN_POINT('',(1.01,-0.505,27.));
#3236=CARTESIAN_POINT('',(1.51,-1.51,27.));
#3237=CARTESIAN_POINT('',(1.51,-1.51,27.));
#3238=CARTESIAN_POINT('',(-1.51,-1.51,27.));
#3239=CARTESIAN_POINT('',(-1.51,-1.51,27.));
#3240=CARTESIAN_POINT('',(-1.51,1.51,27.));
#3241=CARTESIAN_POINT('',(-1.51,1.51,27.));
#3242=CARTESIAN_POINT('',(1.51,1.51,27.));
#3243=CARTESIAN_POINT('',(1.51,1.51,27.));
#3244=CARTESIAN_POINT('',(1.51,-1.51,27.));
#3245=CARTESIAN_POINT('Origin',(1.01,-1.01,26.9));
#3246=CARTESIAN_POINT('',(1.01,-1.01,29.));
#3247=CARTESIAN_POINT('',(1.01,-1.01,26.9));
#3248=CARTESIAN_POINT('',(1.01,-0.505,29.));
#3249=CARTESIAN_POINT('Origin',(1.01,-1.01,26.9));
#3250=CARTESIAN_POINT('',(1.01,1.01,29.));
#3251=CARTESIAN_POINT('',(1.01,-0.505,29.));
#3252=CARTESIAN_POINT('',(1.01,1.01,26.9));
#3253=CARTESIAN_POINT('Origin',(2.2,-1.8,26.));
#3254=CARTESIAN_POINT('',(2.2,-1.8,29.));
#3255=CARTESIAN_POINT('',(2.2,-1.8,29.));
#3256=CARTESIAN_POINT('',(2.2,-1.8,26.));
#3257=CARTESIAN_POINT('',(2.2,-1.8,26.));
#3258=CARTESIAN_POINT('',(2.2,1.8,26.));
#3259=CARTESIAN_POINT('',(2.2,-1.8,26.));
#3260=CARTESIAN_POINT('',(2.2,1.8,29.));
#3261=CARTESIAN_POINT('',(2.2,1.8,26.));
#3262=CARTESIAN_POINT('',(2.2,-1.8,29.));
#3263=CARTESIAN_POINT('Origin',(0.,0.,29.));
#3264=CARTESIAN_POINT('',(-2.2,1.8,29.));
#3265=CARTESIAN_POINT('',(2.2,1.8,29.));
#3266=CARTESIAN_POINT('',(-2.2,-1.8,29.));
#3267=CARTESIAN_POINT('',(-2.2,1.8,29.));
#3268=CARTESIAN_POINT('',(-2.2,-1.8,29.));
#3269=CARTESIAN_POINT('',(-1.01,-1.01,29.));
#3270=CARTESIAN_POINT('',(-0.505,-1.01,29.));
#3271=CARTESIAN_POINT('',(-1.01,1.01,29.));
#3272=CARTESIAN_POINT('',(-1.01,0.505,29.));
#3273=CARTESIAN_POINT('',(0.505,1.01,29.));
#3274=CARTESIAN_POINT('Origin',(-1.01,-1.01,26.9));
#3275=CARTESIAN_POINT('',(-1.01,-1.01,26.9));
#3276=CARTESIAN_POINT('Origin',(1.01,1.01,26.9));
#3277=CARTESIAN_POINT('',(-1.01,1.01,26.9));
#3278=CARTESIAN_POINT('Origin',(-1.01,1.01,26.9));
#3279=CARTESIAN_POINT('Origin',(-1.51,-1.51,25.9));
#3280=CARTESIAN_POINT('',(-1.51,-1.51,26.));
#3281=CARTESIAN_POINT('',(1.51,-1.51,26.));
#3282=CARTESIAN_POINT('',(-0.755,-1.51,26.));
#3283=CARTESIAN_POINT('',(-1.51,-1.51,25.9));
#3284=CARTESIAN_POINT('',(1.51,-1.51,25.9));
#3285=CARTESIAN_POINT('Origin',(1.51,-1.51,25.9));
#3286=CARTESIAN_POINT('',(1.51,1.51,26.));
#3287=CARTESIAN_POINT('',(1.51,-0.755,26.));
#3288=CARTESIAN_POINT('',(1.51,1.51,25.9));
#3289=CARTESIAN_POINT('Origin',(1.51,1.51,25.9));
#3290=CARTESIAN_POINT('',(-1.51,1.51,26.));
#3291=CARTESIAN_POINT('',(0.755,1.51,26.));
#3292=CARTESIAN_POINT('',(-1.51,1.51,25.9));
#3293=CARTESIAN_POINT('Origin',(-1.51,1.51,25.9));
#3294=CARTESIAN_POINT('',(-1.51,0.755,26.));
#3295=CARTESIAN_POINT('Origin',(2.2,1.8,26.));
#3296=CARTESIAN_POINT('',(-2.2,1.8,26.));
#3297=CARTESIAN_POINT('',(2.2,1.8,26.));
#3298=CARTESIAN_POINT('',(-2.2,1.8,26.));
#3299=CARTESIAN_POINT('Origin',(-2.2,-1.8,26.));
#3300=CARTESIAN_POINT('',(-2.2,-1.8,26.));
#3301=CARTESIAN_POINT('',(-2.2,-1.8,26.));
#3302=CARTESIAN_POINT('',(-2.2,-1.8,26.));
#3303=CARTESIAN_POINT('Origin',(-2.2,1.8,26.));
#3304=CARTESIAN_POINT('',(-2.2,1.8,26.));
#3305=CARTESIAN_POINT('Origin',(0.,0.,26.));
#3752=UNCERTAINTY_MEASURE_WITH_UNIT(LENGTH_MEASURE(0.001),#3774,
'DISTANCE_ACCURACY_VALUE',
'Maximum model space distance between geometric entities at asserted c
onnectivities');
#3760=UNCERTAINTY_MEASURE_WITH_UNIT(LENGTH_MEASURE(0.001),#3774,
'DISTANCE_ACCURACY_VALUE',
'Maximum model space distance between geometric entities at asserted c
onnectivities');
#3765=(
GEOMETRIC_REPRESENTATION_CONTEXT(3)
GLOBAL_UNCERTAINTY_ASSIGNED_CONTEXT((#3752))
GLOBAL_UNIT_ASSIGNED_CONTEXT((#3774,#3776,#3777))
REPRESENTATION_CONTEXT('','3D')
);
#3773=(
GEOMETRIC_REPRESENTATION_CONTEXT(3)
GLOBAL_UNCERTAINTY_ASSIGNED_CONTEXT((#3760))
GLOBAL_UNIT_ASSIGNED_CONTEXT((#3774,#3776,#3777))
REPRESENTATION_CONTEXT('','3D')
);
#3774=(
LENGTH_UNIT()
NAMED_UNIT(*)
SI_UNIT(.CENTI.,.METRE.)
);
#3776=(
NAMED_UNIT(*)
PLANE_ANGLE_UNIT()
SI_UNIT($,.RADIAN.)
);
#3777=(
NAMED_UNIT(*)
SI_UNIT($,.STERADIAN.)
SOLID_ANGLE_UNIT()
);
#3782=SHAPE_DEFINITION_REPRESENTATION(#3794,#3817);
#3794=PRODUCT_DEFINITION_SHAPE('',$,#3830);
#3817=SHAPE_REPRESENTATION('',(#2357),#3765);
#3825=PRODUCT_DEFINITION_CONTEXT('part definition',#3863,'design');
#3830=PRODUCT_DEFINITION('Split clamp block','Split clamp block',
#3842,#3825);
#3842=PRODUCT_DEFINITION_FORMATION('',$,#3869);
#3863=APPLICATION_CONTEXT(
'Core Data for Automotive Mechanical Design Process');
#3864=PRODUCT_CONTEXT('part definition',#3863,'mechanical');
#3869=PRODUCT('Split clamp block','Split clamp block',
'Split clamp block',(#3864));
#3919=COLOUR_RGB('Dark Blue',0.08,0.2,0.34);
#3920=FILL_AREA_STYLE_COLOUR('',#3919);
#3921=FILL_AREA_STYLE('',(#3920));
#3922=SURFACE_STYLE_FILL_AREA(#3921);
#3923=SURFACE_SIDE_STYLE('',(#3922));
#3924=SURFACE_STYLE_USAGE(.BOTH.,#3923);
#3925=PRESENTATION_STYLE_ASSIGNMENT((#3924));
ENDSEC;
END-ISO-10303-21;
